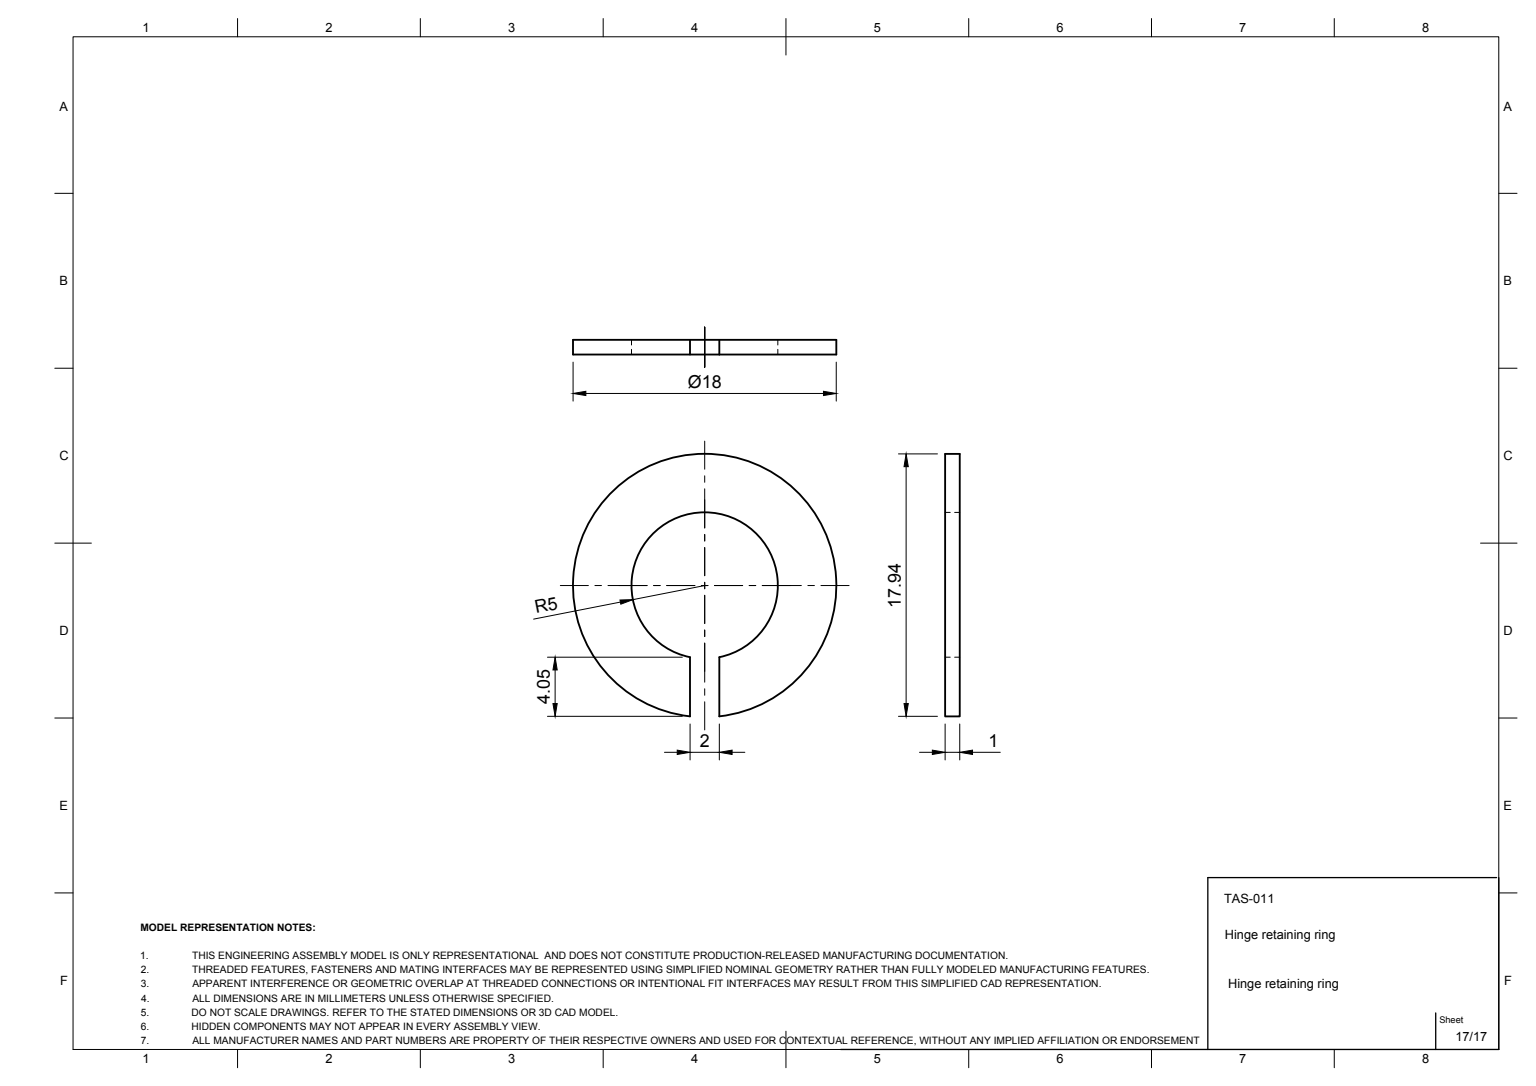
ISO-10303-21;
HEADER;
/* Generated by software containing ST-Developer
 * from STEP Tools, Inc. (www.steptools.com) 
 */

FILE_DESCRIPTION(
/* description */ (
'Independent manual bench leaf bending machine,200mm work width. Fabri
cated welded frame and folding leaf, repeated bushed and fully retaine
d hinge hardware, two handles with bonded grips, beveled clamping beam
 and modeledM12 clamp screws.2mm omitted-workpiece assembly reference 
gap, not a capacity claim. Native135deg hinge travel. Weld sizing, pro
duction fits, material condition, bending capacity, strength and life 
unassigned.'),
/* implementation_level */ '2;1');

FILE_NAME(
/* name */ 'Hinge retaining ring.step',
/* time_stamp */ '2026-11-14T09:11:34-08:00',
/* author */ (''),
/* organization */ (''),
/* preprocessor_version */ 'ST-DEVELOPER v20.2',
/* originating_system */ 'Autodesk Translation Framework v15.17.0.0',
/* authorisation */ '');

FILE_SCHEMA (('AUTOMOTIVE_DESIGN { 1 0 10303 214 3 1 1 }'));
ENDSEC;

DATA;
#10=MECHANICAL_DESIGN_GEOMETRIC_PRESENTATION_REPRESENTATION('',(#463),#37701);
#427=SHAPE_REPRESENTATION_RELATIONSHIP('SRR','None',#37796,#445);
#445=ADVANCED_BREP_SHAPE_REPRESENTATION('',(#481),#37700);
#463=STYLED_ITEM('',(#37883),#481);
#481=MANIFOLD_SOLID_BREP('Body1',#4161);
#598=PLANE('',#4663);
#599=PLANE('',#4664);
#600=PLANE('',#4665);
#601=PLANE('',#4672);
#808=FACE_OUTER_BOUND('',#1054,.T.);
#809=FACE_OUTER_BOUND('',#1055,.T.);
#810=FACE_OUTER_BOUND('',#1056,.T.);
#811=FACE_OUTER_BOUND('',#1057,.T.);
#812=FACE_OUTER_BOUND('',#1058,.T.);
#813=FACE_OUTER_BOUND('',#1059,.T.);
#1054=EDGE_LOOP('',(#3787,#3788,#3789,#3790));
#1055=EDGE_LOOP('',(#3791,#3792,#3793,#3794));
#1056=EDGE_LOOP('',(#3795,#3796,#3797,#3798));
#1057=EDGE_LOOP('',(#3799,#3800,#3801,#3802));
#1058=EDGE_LOOP('',(#3803,#3804,#3805,#3806));
#1059=EDGE_LOOP('',(#3807,#3808,#3809,#3810));
#1301=LINE('',#37605,#1550);
#1302=LINE('',#37607,#1551);
#1303=LINE('',#37609,#1552);
#1304=LINE('',#37610,#1553);
#1305=LINE('',#37614,#1554);
#1306=LINE('',#37616,#1555);
#1307=LINE('',#37618,#1556);
#1308=LINE('',#37619,#1557);
#1550=VECTOR('',#5554,10.);
#1551=VECTOR('',#5555,10.);
#1552=VECTOR('',#5556,10.);
#1553=VECTOR('',#5557,10.);
#1554=VECTOR('',#5560,10.);
#1555=VECTOR('',#5561,10.);
#1556=VECTOR('',#5562,10.);
#1557=VECTOR('',#5563,10.);
#1633=CIRCLE('',#4666,9.);
#1634=CIRCLE('',#4667,5.);
#1635=CIRCLE('',#4669,5.);
#1636=CIRCLE('',#4671,9.);
#2045=VERTEX_POINT('',#37603);
#2046=VERTEX_POINT('',#37604);
#2047=VERTEX_POINT('',#37606);
#2048=VERTEX_POINT('',#37608);
#2049=VERTEX_POINT('',#37612);
#2050=VERTEX_POINT('',#37613);
#2051=VERTEX_POINT('',#37615);
#2052=VERTEX_POINT('',#37617);
#2627=EDGE_CURVE('',#2045,#2046,#1301,.T.);
#2628=EDGE_CURVE('',#2047,#2045,#1302,.T.);
#2629=EDGE_CURVE('',#2048,#2047,#1303,.T.);
#2630=EDGE_CURVE('',#2046,#2048,#1304,.T.);
#2631=EDGE_CURVE('',#2049,#2050,#1305,.T.);
#2632=EDGE_CURVE('',#2051,#2049,#1306,.T.);
#2633=EDGE_CURVE('',#2052,#2051,#1307,.T.);
#2634=EDGE_CURVE('',#2050,#2052,#1308,.T.);
#2635=EDGE_CURVE('',#2047,#2052,#1633,.T.);
#2636=EDGE_CURVE('',#2050,#2045,#1634,.T.);
#2637=EDGE_CURVE('',#2049,#2046,#1635,.T.);
#2638=EDGE_CURVE('',#2048,#2051,#1636,.T.);
#3787=ORIENTED_EDGE('',*,*,#2627,.F.);
#3788=ORIENTED_EDGE('',*,*,#2628,.F.);
#3789=ORIENTED_EDGE('',*,*,#2629,.F.);
#3790=ORIENTED_EDGE('',*,*,#2630,.F.);
#3791=ORIENTED_EDGE('',*,*,#2631,.F.);
#3792=ORIENTED_EDGE('',*,*,#2632,.F.);
#3793=ORIENTED_EDGE('',*,*,#2633,.F.);
#3794=ORIENTED_EDGE('',*,*,#2634,.F.);
#3795=ORIENTED_EDGE('',*,*,#2634,.T.);
#3796=ORIENTED_EDGE('',*,*,#2635,.F.);
#3797=ORIENTED_EDGE('',*,*,#2628,.T.);
#3798=ORIENTED_EDGE('',*,*,#2636,.F.);
#3799=ORIENTED_EDGE('',*,*,#2631,.T.);
#3800=ORIENTED_EDGE('',*,*,#2636,.T.);
#3801=ORIENTED_EDGE('',*,*,#2627,.T.);
#3802=ORIENTED_EDGE('',*,*,#2637,.F.);
#3803=ORIENTED_EDGE('',*,*,#2633,.T.);
#3804=ORIENTED_EDGE('',*,*,#2638,.F.);
#3805=ORIENTED_EDGE('',*,*,#2629,.T.);
#3806=ORIENTED_EDGE('',*,*,#2635,.T.);
#3807=ORIENTED_EDGE('',*,*,#2632,.T.);
#3808=ORIENTED_EDGE('',*,*,#2637,.T.);
#3809=ORIENTED_EDGE('',*,*,#2630,.T.);
#3810=ORIENTED_EDGE('',*,*,#2638,.T.);
#3930=CYLINDRICAL_SURFACE('',#4668,5.);
#3931=CYLINDRICAL_SURFACE('',#4670,9.);
#4138=ADVANCED_FACE('',(#808),#598,.F.);
#4139=ADVANCED_FACE('',(#809),#599,.F.);
#4140=ADVANCED_FACE('',(#810),#600,.F.);
#4141=ADVANCED_FACE('',(#811),#3930,.F.);
#4142=ADVANCED_FACE('',(#812),#3931,.T.);
#4143=ADVANCED_FACE('',(#813),#601,.T.);
#4161=CLOSED_SHELL('',(#4138,#4139,#4140,#4141,#4142,#4143));
#4662=AXIS2_PLACEMENT_3D('',#37601,#5550,#5551);
#4663=AXIS2_PLACEMENT_3D('',#37602,#5552,#5553);
#4664=AXIS2_PLACEMENT_3D('',#37611,#5558,#5559);
#4665=AXIS2_PLACEMENT_3D('',#37620,#5564,#5565);
#4666=AXIS2_PLACEMENT_3D('',#37621,#5566,#5567);
#4667=AXIS2_PLACEMENT_3D('',#37622,#5568,#5569);
#4668=AXIS2_PLACEMENT_3D('',#37623,#5570,#5571);
#4669=AXIS2_PLACEMENT_3D('',#37624,#5572,#5573);
#4670=AXIS2_PLACEMENT_3D('',#37625,#5574,#5575);
#4671=AXIS2_PLACEMENT_3D('',#37626,#5576,#5577);
#4672=AXIS2_PLACEMENT_3D('',#37627,#5578,#5579);
#5550=DIRECTION('axis',(0.,0.,1.));
#5551=DIRECTION('refdir',(1.,0.,0.));
#5552=DIRECTION('center_axis',(-1.,0.,0.));
#5553=DIRECTION('ref_axis',(0.,1.,0.));
#5554=DIRECTION('',(0.,0.,1.));
#5555=DIRECTION('',(0.,-1.,0.));
#5556=DIRECTION('',(0.,0.,-1.));
#5557=DIRECTION('',(0.,1.,0.));
#5558=DIRECTION('center_axis',(1.,0.,0.));
#5559=DIRECTION('ref_axis',(0.,-1.,0.));
#5560=DIRECTION('',(0.,0.,-1.));
#5561=DIRECTION('',(0.,-1.,0.));
#5562=DIRECTION('',(0.,0.,1.));
#5563=DIRECTION('',(0.,1.,0.));
#5564=DIRECTION('center_axis',(0.,0.,1.));
#5565=DIRECTION('ref_axis',(1.,0.,0.));
#5566=DIRECTION('center_axis',(0.,0.,1.));
#5567=DIRECTION('ref_axis',(1.,0.,0.));
#5568=DIRECTION('center_axis',(0.,0.,-1.));
#5569=DIRECTION('ref_axis',(1.,0.,0.));
#5570=DIRECTION('center_axis',(0.,0.,1.));
#5571=DIRECTION('ref_axis',(6.12323399573677E-17,-1.,0.));
#5572=DIRECTION('center_axis',(0.,0.,-1.));
#5573=DIRECTION('ref_axis',(1.,0.,0.));
#5574=DIRECTION('center_axis',(0.,0.,1.));
#5575=DIRECTION('ref_axis',(6.12323399573677E-17,-1.,0.));
#5576=DIRECTION('center_axis',(0.,0.,1.));
#5577=DIRECTION('ref_axis',(1.,0.,0.));
#5578=DIRECTION('center_axis',(0.,0.,1.));
#5579=DIRECTION('ref_axis',(1.,0.,0.));
#37601=CARTESIAN_POINT('',(0.,0.,0.));
#37602=CARTESIAN_POINT('Origin',(-1.,0.,1.));
#37603=CARTESIAN_POINT('',(-1.,4.89897948556636,0.));
#37604=CARTESIAN_POINT('',(-1.,4.89897948556636,1.));
#37605=CARTESIAN_POINT('',(-1.,4.89897948556636,0.));
#37606=CARTESIAN_POINT('',(-1.,8.94427190999916,0.));
#37607=CARTESIAN_POINT('',(-1.,0.,0.));
#37608=CARTESIAN_POINT('',(-1.,8.94427190999916,1.));
#37609=CARTESIAN_POINT('',(-1.,8.94427190999916,0.));
#37610=CARTESIAN_POINT('',(-1.,0.,1.));
#37611=CARTESIAN_POINT('Origin',(1.,18.,1.));
#37612=CARTESIAN_POINT('',(1.,4.89897948556636,1.));
#37613=CARTESIAN_POINT('',(1.,4.89897948556636,0.));
#37614=CARTESIAN_POINT('',(1.,4.89897948556636,0.));
#37615=CARTESIAN_POINT('',(1.,8.94427190999916,1.));
#37616=CARTESIAN_POINT('',(1.,9.,1.));
#37617=CARTESIAN_POINT('',(1.,8.94427190999916,0.));
#37618=CARTESIAN_POINT('',(1.,8.94427190999916,0.));
#37619=CARTESIAN_POINT('',(1.,9.,0.));
#37620=CARTESIAN_POINT('Origin',(0.,0.,0.));
#37621=CARTESIAN_POINT('Origin',(0.,0.,0.));
#37622=CARTESIAN_POINT('Origin',(0.,0.,0.));
#37623=CARTESIAN_POINT('Origin',(0.,0.,0.));
#37624=CARTESIAN_POINT('Origin',(0.,0.,1.));
#37625=CARTESIAN_POINT('Origin',(0.,0.,0.));
#37626=CARTESIAN_POINT('Origin',(0.,0.,1.));
#37627=CARTESIAN_POINT('Origin',(0.,0.,1.));
#37680=UNCERTAINTY_MEASURE_WITH_UNIT(LENGTH_MEASURE(0.01),#37702,
'DISTANCE_ACCURACY_VALUE',
'Maximum model space distance between geometric entities at asserted c
onnectivities');
#37681=UNCERTAINTY_MEASURE_WITH_UNIT(LENGTH_MEASURE(0.01),#37702,
'DISTANCE_ACCURACY_VALUE',
'Maximum model space distance between geometric entities at asserted c
onnectivities');
#37700=(
GEOMETRIC_REPRESENTATION_CONTEXT(3)
GLOBAL_UNCERTAINTY_ASSIGNED_CONTEXT((#37680))
GLOBAL_UNIT_ASSIGNED_CONTEXT((#37702,#37704,#37705))
REPRESENTATION_CONTEXT('','3D')
);
#37701=(
GEOMETRIC_REPRESENTATION_CONTEXT(3)
GLOBAL_UNCERTAINTY_ASSIGNED_CONTEXT((#37681))
GLOBAL_UNIT_ASSIGNED_CONTEXT((#37702,#37704,#37705))
REPRESENTATION_CONTEXT('','3D')
);
#37702=(
LENGTH_UNIT()
NAMED_UNIT(*)
SI_UNIT(.MILLI.,.METRE.)
);
#37704=(
NAMED_UNIT(*)
PLANE_ANGLE_UNIT()
SI_UNIT($,.RADIAN.)
);
#37705=(
NAMED_UNIT(*)
SI_UNIT($,.STERADIAN.)
SOLID_ANGLE_UNIT()
);
#37724=SHAPE_DEFINITION_REPRESENTATION(#37743,#37796);
#37743=PRODUCT_DEFINITION_SHAPE('',$,#37816);
#37796=SHAPE_REPRESENTATION('',(#4662),#37700);
#37797=PRODUCT_DEFINITION_CONTEXT('part definition',#37856,'design');
#37816=PRODUCT_DEFINITION('Hinge retaining ring','Hinge retaining ring',
#37835,#37797);
#37835=PRODUCT_DEFINITION_FORMATION('',$,#37876);
#37856=APPLICATION_CONTEXT(
'Core Data for Automotive Mechanical Design Process');
#37857=PRODUCT_CONTEXT('part definition',#37856,'mechanical');
#37876=PRODUCT('Hinge retaining ring','Hinge retaining ring',$,(#37857));
#37883=PRESENTATION_STYLE_ASSIGNMENT((#37891));
#37891=SURFACE_STYLE_USAGE(.BOTH.,#37899);
#37899=SURFACE_SIDE_STYLE('',(#37907));
#37907=SURFACE_STYLE_FILL_AREA(#37915);
#37915=FILL_AREA_STYLE('Opaque(64,72,82)',(#37923));
#37923=FILL_AREA_STYLE_COLOUR('Opaque(64,72,82)',#37931);
#37931=COLOUR_RGB('Opaque(64,72,82)',0.250980392156863,0.282352941176471,
0.32156862745098);
ENDSEC;
END-ISO-10303-21;
